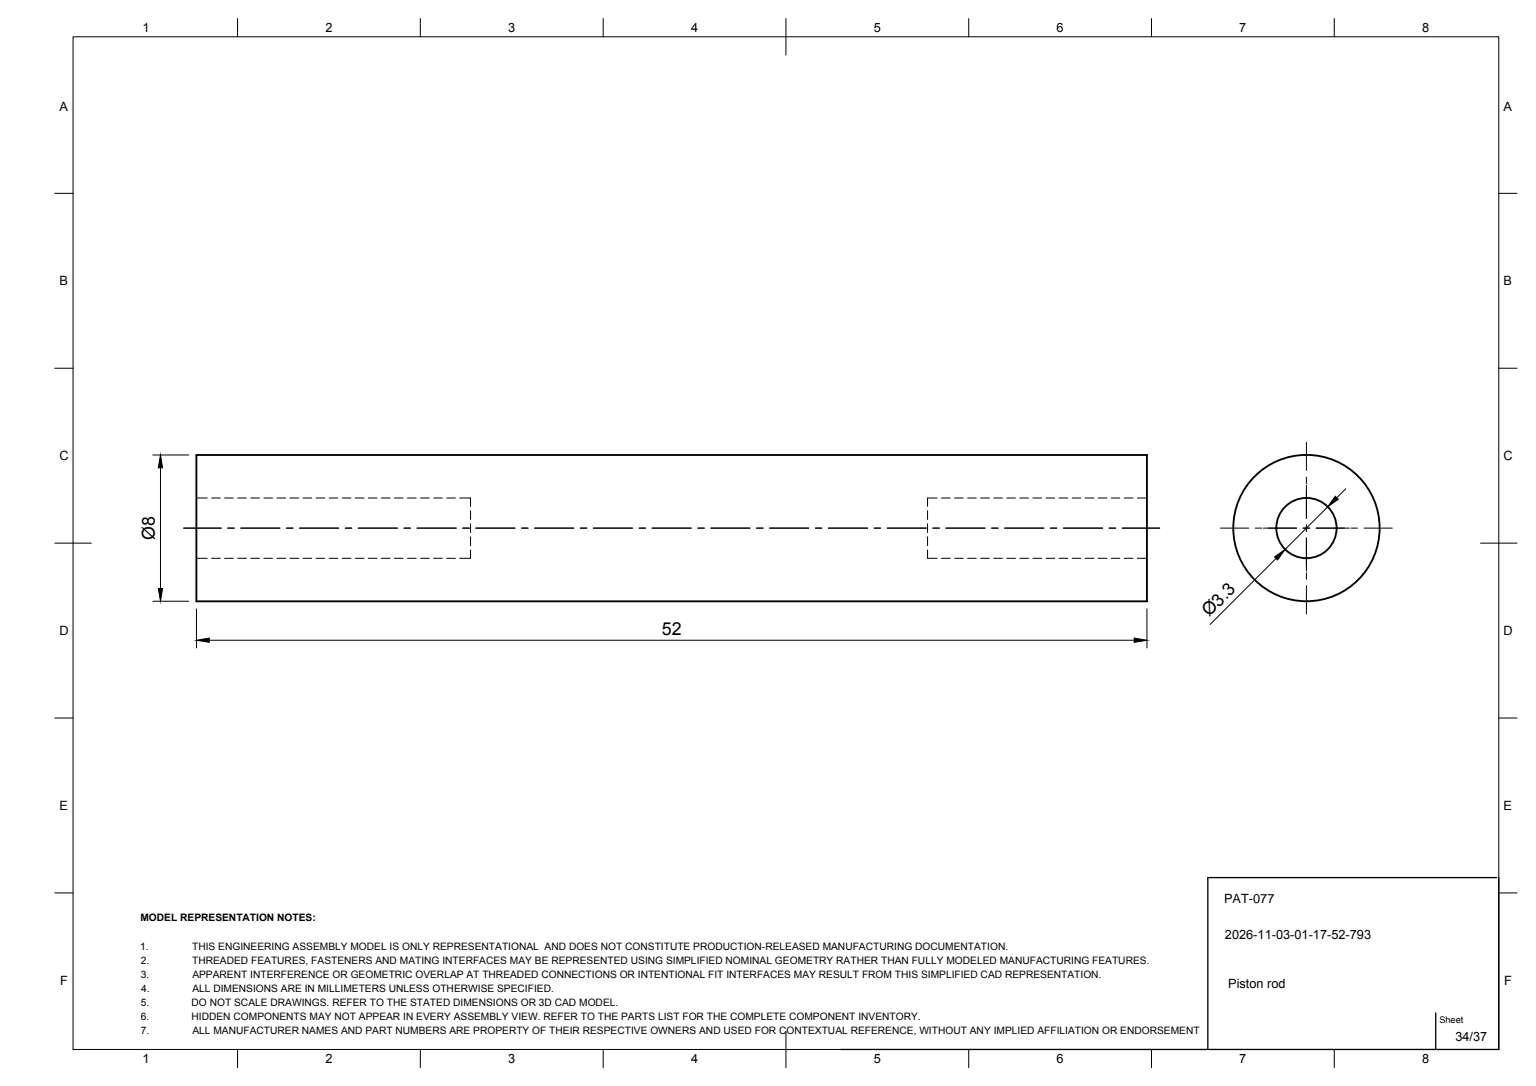
ISO-10303-21;
HEADER;
/* Generated by software containing ST-Developer
 * from STEP Tools, Inc. (www.steptools.com) 
 */

FILE_DESCRIPTION(
/* description */ ('Pallet stop with pneumatic fitting'),
/* implementation_level */ '2;1');

FILE_NAME(
/* name */ 'Piston rod.step',
/* time_stamp */ '2026-10-27T10:51:41-07:00',
/* author */ (''),
/* organization */ (''),
/* preprocessor_version */ 'ST-DEVELOPER v20.2',
/* originating_system */ 'Autodesk Translation Framework v15.17.0.0',
/* authorisation */ '');

FILE_SCHEMA (('AUTOMOTIVE_DESIGN { 1 0 10303 214 3 1 1 }'));
ENDSEC;

DATA;
#10=MECHANICAL_DESIGN_GEOMETRIC_PRESENTATION_REPRESENTATION('',(#383),#10265);
#319=SHAPE_REPRESENTATION_RELATIONSHIP('SRR','None',#10435,#351);
#351=ADVANCED_BREP_SHAPE_REPRESENTATION('',(#414),#10259);
#383=STYLED_ITEM('',(#10655),#414);
#414=MANIFOLD_SOLID_BREP('Body1',#5072);
#535=FACE_BOUND('',#1435,.T.);
#536=FACE_BOUND('',#1437,.T.);
#704=PLANE('',#5948);
#705=PLANE('',#5952);
#706=PLANE('',#5956);
#707=PLANE('',#5957);
#999=FACE_OUTER_BOUND('',#1429,.T.);
#1000=FACE_OUTER_BOUND('',#1430,.T.);
#1001=FACE_OUTER_BOUND('',#1431,.T.);
#1002=FACE_OUTER_BOUND('',#1432,.T.);
#1003=FACE_OUTER_BOUND('',#1433,.T.);
#1004=FACE_OUTER_BOUND('',#1434,.T.);
#1005=FACE_OUTER_BOUND('',#1436,.T.);
#1429=EDGE_LOOP('',(#4448,#4449,#4450,#4451));
#1430=EDGE_LOOP('',(#4452));
#1431=EDGE_LOOP('',(#4453,#4454,#4455,#4456));
#1432=EDGE_LOOP('',(#4457));
#1433=EDGE_LOOP('',(#4458,#4459,#4460,#4461));
#1434=EDGE_LOOP('',(#4462));
#1435=EDGE_LOOP('',(#4463));
#1436=EDGE_LOOP('',(#4464));
#1437=EDGE_LOOP('',(#4465));
#1770=LINE('',#9939,#2105);
#1771=LINE('',#9946,#2106);
#1772=LINE('',#9953,#2107);
#2105=VECTOR('',#7399,0.165);
#2106=VECTOR('',#7408,0.165);
#2107=VECTOR('',#7417,0.4);
#2375=CIRCLE('',#5946,0.165);
#2376=CIRCLE('',#5947,0.165);
#2377=CIRCLE('',#5950,0.165);
#2378=CIRCLE('',#5951,0.165);
#2379=CIRCLE('',#5954,0.4);
#2380=CIRCLE('',#5955,0.4);
#2748=VERTEX_POINT('',#9936);
#2749=VERTEX_POINT('',#9938);
#2750=VERTEX_POINT('',#9943);
#2751=VERTEX_POINT('',#9945);
#2752=VERTEX_POINT('',#9950);
#2753=VERTEX_POINT('',#9952);
#3323=EDGE_CURVE('',#2748,#2748,#2375,.T.);
#3324=EDGE_CURVE('',#2748,#2749,#1770,.T.);
#3325=EDGE_CURVE('',#2749,#2749,#2376,.T.);
#3326=EDGE_CURVE('',#2750,#2750,#2377,.T.);
#3327=EDGE_CURVE('',#2750,#2751,#1771,.T.);
#3328=EDGE_CURVE('',#2751,#2751,#2378,.T.);
#3329=EDGE_CURVE('',#2752,#2752,#2379,.T.);
#3330=EDGE_CURVE('',#2752,#2753,#1772,.T.);
#3331=EDGE_CURVE('',#2753,#2753,#2380,.T.);
#4448=ORIENTED_EDGE('',*,*,#3323,.F.);
#4449=ORIENTED_EDGE('',*,*,#3324,.T.);
#4450=ORIENTED_EDGE('',*,*,#3325,.F.);
#4451=ORIENTED_EDGE('',*,*,#3324,.F.);
#4452=ORIENTED_EDGE('',*,*,#3323,.T.);
#4453=ORIENTED_EDGE('',*,*,#3326,.F.);
#4454=ORIENTED_EDGE('',*,*,#3327,.T.);
#4455=ORIENTED_EDGE('',*,*,#3328,.T.);
#4456=ORIENTED_EDGE('',*,*,#3327,.F.);
#4457=ORIENTED_EDGE('',*,*,#3328,.F.);
#4458=ORIENTED_EDGE('',*,*,#3329,.F.);
#4459=ORIENTED_EDGE('',*,*,#3330,.T.);
#4460=ORIENTED_EDGE('',*,*,#3331,.T.);
#4461=ORIENTED_EDGE('',*,*,#3330,.F.);
#4462=ORIENTED_EDGE('',*,*,#3329,.T.);
#4463=ORIENTED_EDGE('',*,*,#3325,.T.);
#4464=ORIENTED_EDGE('',*,*,#3331,.F.);
#4465=ORIENTED_EDGE('',*,*,#3326,.T.);
#4718=CYLINDRICAL_SURFACE('',#5945,0.165);
#4719=CYLINDRICAL_SURFACE('',#5949,0.165);
#4720=CYLINDRICAL_SURFACE('',#5953,0.4);
#4994=ADVANCED_FACE('',(#999),#4718,.F.);
#4995=ADVANCED_FACE('',(#1000),#704,.T.);
#4996=ADVANCED_FACE('',(#1001),#4719,.F.);
#4997=ADVANCED_FACE('',(#1002),#705,.F.);
#4998=ADVANCED_FACE('',(#1003),#4720,.T.);
#4999=ADVANCED_FACE('',(#1004,#535),#706,.T.);
#5000=ADVANCED_FACE('',(#1005,#536),#707,.F.);
#5072=CLOSED_SHELL('',(#4994,#4995,#4996,#4997,#4998,#4999,#5000));
#5944=AXIS2_PLACEMENT_3D('',#9934,#7393,#7394);
#5945=AXIS2_PLACEMENT_3D('',#9935,#7395,#7396);
#5946=AXIS2_PLACEMENT_3D('',#9937,#7397,#7398);
#5947=AXIS2_PLACEMENT_3D('',#9940,#7400,#7401);
#5948=AXIS2_PLACEMENT_3D('',#9941,#7402,#7403);
#5949=AXIS2_PLACEMENT_3D('',#9942,#7404,#7405);
#5950=AXIS2_PLACEMENT_3D('',#9944,#7406,#7407);
#5951=AXIS2_PLACEMENT_3D('',#9947,#7409,#7410);
#5952=AXIS2_PLACEMENT_3D('',#9948,#7411,#7412);
#5953=AXIS2_PLACEMENT_3D('',#9949,#7413,#7414);
#5954=AXIS2_PLACEMENT_3D('',#9951,#7415,#7416);
#5955=AXIS2_PLACEMENT_3D('',#9954,#7418,#7419);
#5956=AXIS2_PLACEMENT_3D('',#9955,#7420,#7421);
#5957=AXIS2_PLACEMENT_3D('',#9956,#7422,#7423);
#7393=DIRECTION('axis',(0.,0.,1.));
#7394=DIRECTION('refdir',(1.,0.,0.));
#7395=DIRECTION('center_axis',(0.,0.,1.));
#7396=DIRECTION('ref_axis',(1.,0.,0.));
#7397=DIRECTION('center_axis',(0.,0.,1.));
#7398=DIRECTION('ref_axis',(1.,0.,0.));
#7399=DIRECTION('',(0.,0.,1.));
#7400=DIRECTION('center_axis',(0.,0.,-1.));
#7401=DIRECTION('ref_axis',(1.,0.,0.));
#7402=DIRECTION('center_axis',(0.,0.,1.));
#7403=DIRECTION('ref_axis',(1.,0.,0.));
#7404=DIRECTION('center_axis',(0.,0.,1.));
#7405=DIRECTION('ref_axis',(1.,0.,0.));
#7406=DIRECTION('center_axis',(0.,0.,1.));
#7407=DIRECTION('ref_axis',(1.,0.,0.));
#7408=DIRECTION('',(0.,0.,1.));
#7409=DIRECTION('center_axis',(0.,0.,1.));
#7410=DIRECTION('ref_axis',(1.,0.,0.));
#7411=DIRECTION('center_axis',(0.,0.,1.));
#7412=DIRECTION('ref_axis',(1.,0.,0.));
#7413=DIRECTION('center_axis',(0.,0.,1.));
#7414=DIRECTION('ref_axis',(1.,0.,0.));
#7415=DIRECTION('center_axis',(0.,0.,1.));
#7416=DIRECTION('ref_axis',(1.,0.,0.));
#7417=DIRECTION('',(0.,0.,-1.));
#7418=DIRECTION('center_axis',(0.,0.,1.));
#7419=DIRECTION('ref_axis',(1.,0.,0.));
#7420=DIRECTION('center_axis',(0.,0.,1.));
#7421=DIRECTION('ref_axis',(1.,0.,0.));
#7422=DIRECTION('center_axis',(0.,0.,1.));
#7423=DIRECTION('ref_axis',(1.,0.,0.));
#9934=CARTESIAN_POINT('',(0.,0.,0.));
#9935=CARTESIAN_POINT('Origin',(4.,4.,11.5));
#9936=CARTESIAN_POINT('',(3.835,4.,11.5));
#9937=CARTESIAN_POINT('Origin',(4.,4.,11.5));
#9938=CARTESIAN_POINT('',(3.835,4.,13.));
#9939=CARTESIAN_POINT('',(3.835,4.,11.5));
#9940=CARTESIAN_POINT('Origin',(4.,4.,13.));
#9941=CARTESIAN_POINT('Origin',(4.,4.,11.5));
#9942=CARTESIAN_POINT('Origin',(4.,4.,7.7));
#9943=CARTESIAN_POINT('',(3.835,4.,7.8));
#9944=CARTESIAN_POINT('Origin',(4.,4.,7.8));
#9945=CARTESIAN_POINT('',(3.835,4.,9.));
#9946=CARTESIAN_POINT('',(3.835,4.,7.7));
#9947=CARTESIAN_POINT('Origin',(4.,4.,9.));
#9948=CARTESIAN_POINT('Origin',(4.,4.,9.));
#9949=CARTESIAN_POINT('Origin',(4.,4.,7.8));
#9950=CARTESIAN_POINT('',(3.6,4.,13.));
#9951=CARTESIAN_POINT('Origin',(4.,4.,13.));
#9952=CARTESIAN_POINT('',(3.6,4.,7.8));
#9953=CARTESIAN_POINT('',(3.6,4.,7.8));
#9954=CARTESIAN_POINT('Origin',(4.,4.,7.8));
#9955=CARTESIAN_POINT('Origin',(4.,4.,13.));
#9956=CARTESIAN_POINT('Origin',(4.,4.,7.8));
#10221=UNCERTAINTY_MEASURE_WITH_UNIT(LENGTH_MEASURE(0.001),#10266,
'DISTANCE_ACCURACY_VALUE',
'Maximum model space distance between geometric entities at asserted c
onnectivities');
#10227=UNCERTAINTY_MEASURE_WITH_UNIT(LENGTH_MEASURE(0.001),#10266,
'DISTANCE_ACCURACY_VALUE',
'Maximum model space distance between geometric entities at asserted c
onnectivities');
#10259=(
GEOMETRIC_REPRESENTATION_CONTEXT(3)
GLOBAL_UNCERTAINTY_ASSIGNED_CONTEXT((#10221))
GLOBAL_UNIT_ASSIGNED_CONTEXT((#10266,#10268,#10269))
REPRESENTATION_CONTEXT('','3D')
);
#10265=(
GEOMETRIC_REPRESENTATION_CONTEXT(3)
GLOBAL_UNCERTAINTY_ASSIGNED_CONTEXT((#10227))
GLOBAL_UNIT_ASSIGNED_CONTEXT((#10266,#10268,#10269))
REPRESENTATION_CONTEXT('','3D')
);
#10266=(
LENGTH_UNIT()
NAMED_UNIT(*)
SI_UNIT(.CENTI.,.METRE.)
);
#10268=(
NAMED_UNIT(*)
PLANE_ANGLE_UNIT()
SI_UNIT($,.RADIAN.)
);
#10269=(
NAMED_UNIT(*)
SI_UNIT($,.STERADIAN.)
SOLID_ANGLE_UNIT()
);
#10301=SHAPE_DEFINITION_REPRESENTATION(#10342,#10435);
#10342=PRODUCT_DEFINITION_SHAPE('',$,#10473);
#10435=SHAPE_REPRESENTATION('',(#5944),#10259);
#10441=PRODUCT_DEFINITION_CONTEXT('part definition',#10554,'design');
#10473=PRODUCT_DEFINITION('Piston rod','Piston rod',#10510,#10441);
#10510=PRODUCT_DEFINITION_FORMATION('',$,#10587);
#10554=APPLICATION_CONTEXT(
'Core Data for Automotive Mechanical Design Process');
#10555=PRODUCT_CONTEXT('part definition',#10554,'mechanical');
#10587=PRODUCT('Piston rod','Piston rod','Piston rod',(#10555));
#10649=COLOUR_RGB('Grey',0.48,0.52,0.57);
#10650=FILL_AREA_STYLE_COLOUR('',#10649);
#10651=FILL_AREA_STYLE('',(#10650));
#10652=SURFACE_STYLE_FILL_AREA(#10651);
#10653=SURFACE_SIDE_STYLE('',(#10652));
#10654=SURFACE_STYLE_USAGE(.BOTH.,#10653);
#10655=PRESENTATION_STYLE_ASSIGNMENT((#10654));
ENDSEC;
END-ISO-10303-21;
